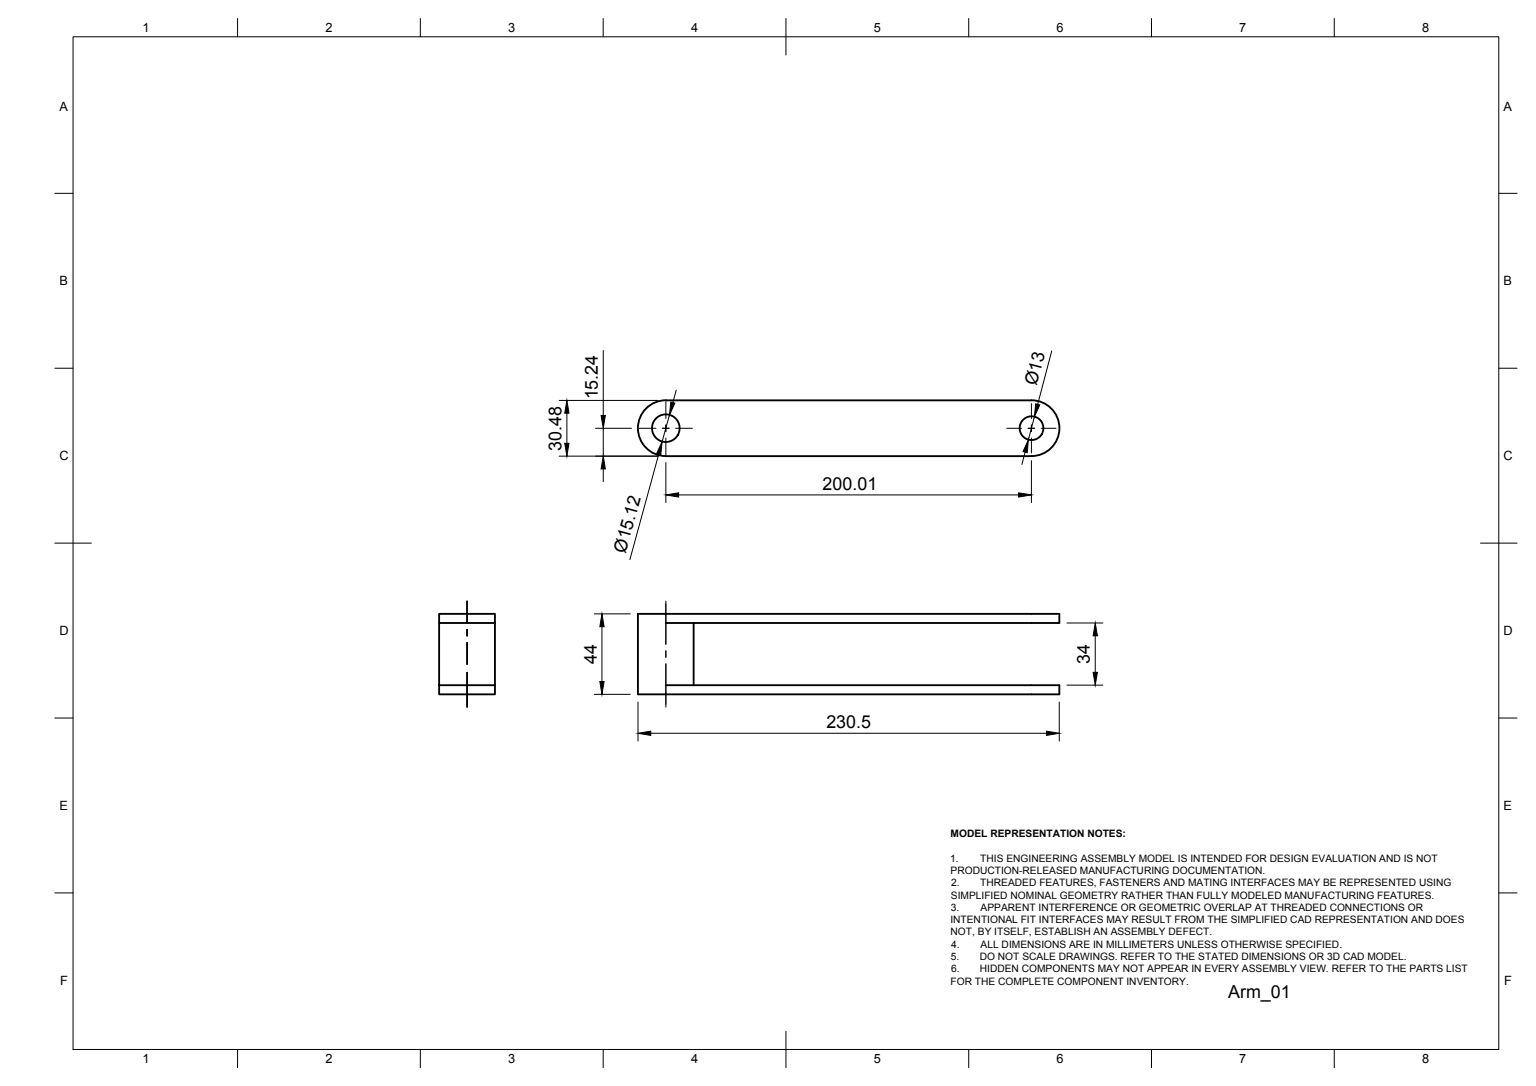
ISO-10303-21;
HEADER;
/* Generated by software containing ST-Developer
 * from STEP Tools, Inc. (www.steptools.com) 
 */

FILE_DESCRIPTION(
/* description */ (''),
/* implementation_level */ '2;1');

FILE_NAME(
/* name */ 'Arm_01.step',
/* time_stamp */ '2026-10-06T13:41:14-07:00',
/* author */ (''),
/* organization */ (''),
/* preprocessor_version */ 'ST-DEVELOPER v20.2',
/* originating_system */ 'Autodesk Translation Framework v15.15.0.0',
/* authorisation */ '');

FILE_SCHEMA (('AUTOMOTIVE_DESIGN { 1 0 10303 214 3 1 1 }'));
ENDSEC;

DATA;
#10=MECHANICAL_DESIGN_GEOMETRIC_PRESENTATION_REPRESENTATION('',(#1964),#279266);
#1946=SHAPE_REPRESENTATION_RELATIONSHIP('SRR','None',#279305,#1955);
#1955=ADVANCED_BREP_SHAPE_REPRESENTATION('',(#1973),#279261);
#1964=STYLED_ITEM('',(#279355),#1973);
#1973=MANIFOLD_SOLID_BREP('Body1',#14942);
#1996=FACE_BOUND('',#2965,.T.);
#1997=FACE_BOUND('',#2967,.T.);
#1998=FACE_BOUND('',#2968,.T.);
#1999=FACE_BOUND('',#2976,.T.);
#2000=FACE_BOUND('',#2978,.T.);
#2001=FACE_BOUND('',#2979,.T.);
#2063=PLANE('',#15478);
#2064=PLANE('',#15482);
#2065=PLANE('',#15483);
#2066=PLANE('',#15485);
#2067=PLANE('',#15493);
#2068=PLANE('',#15497);
#2069=PLANE('',#15501);
#2070=PLANE('',#15502);
#2472=FACE_OUTER_BOUND('',#2960,.T.);
#2473=FACE_OUTER_BOUND('',#2961,.T.);
#2474=FACE_OUTER_BOUND('',#2962,.T.);
#2475=FACE_OUTER_BOUND('',#2963,.T.);
#2476=FACE_OUTER_BOUND('',#2964,.T.);
#2477=FACE_OUTER_BOUND('',#2966,.T.);
#2478=FACE_OUTER_BOUND('',#2969,.T.);
#2479=FACE_OUTER_BOUND('',#2970,.T.);
#2480=FACE_OUTER_BOUND('',#2971,.T.);
#2481=FACE_OUTER_BOUND('',#2972,.T.);
#2482=FACE_OUTER_BOUND('',#2973,.T.);
#2483=FACE_OUTER_BOUND('',#2974,.T.);
#2484=FACE_OUTER_BOUND('',#2975,.T.);
#2485=FACE_OUTER_BOUND('',#2977,.T.);
#2960=EDGE_LOOP('',(#13374,#13375,#13376,#13377));
#2961=EDGE_LOOP('',(#13378,#13379,#13380,#13381));
#2962=EDGE_LOOP('',(#13382,#13383,#13384,#13385));
#2963=EDGE_LOOP('',(#13386,#13387,#13388,#13389));
#2964=EDGE_LOOP('',(#13390,#13391,#13392,#13393));
#2965=EDGE_LOOP('',(#13394));
#2966=EDGE_LOOP('',(#13395,#13396,#13397,#13398));
#2967=EDGE_LOOP('',(#13399));
#2968=EDGE_LOOP('',(#13400));
#2969=EDGE_LOOP('',(#13401,#13402,#13403,#13404));
#2970=EDGE_LOOP('',(#13405,#13406,#13407,#13408));
#2971=EDGE_LOOP('',(#13409,#13410,#13411,#13412));
#2972=EDGE_LOOP('',(#13413,#13414,#13415,#13416));
#2973=EDGE_LOOP('',(#13417,#13418,#13419,#13420));
#2974=EDGE_LOOP('',(#13421,#13422,#13423,#13424,#13425,#13426,#13427,#13428,
#13429,#13430));
#2975=EDGE_LOOP('',(#13431,#13432,#13433,#13434));
#2976=EDGE_LOOP('',(#13435));
#2977=EDGE_LOOP('',(#13436,#13437,#13438,#13439));
#2978=EDGE_LOOP('',(#13440));
#2979=EDGE_LOOP('',(#13441));
#3479=LINE('',#240456,#4007);
#3480=LINE('',#240461,#4008);
#3481=LINE('',#240463,#4009);
#3482=LINE('',#240465,#4010);
#3483=LINE('',#240466,#4011);
#3484=LINE('',#240471,#4012);
#3485=LINE('',#240475,#4013);
#3486=LINE('',#240477,#4014);
#3487=LINE('',#240478,#4015);
#3488=LINE('',#240488,#4016);
#3489=LINE('',#240493,#4017);
#3490=LINE('',#240498,#4018);
#3491=LINE('',#240500,#4019);
#3492=LINE('',#240502,#4020);
#3493=LINE('',#240503,#4021);
#3494=LINE('',#240509,#4022);
#3495=LINE('',#240512,#4023);
#3496=LINE('',#240514,#4024);
#3497=LINE('',#240515,#4025);
#3498=LINE('',#240517,#4026);
#4007=VECTOR('',#16917,6.50110764916953);
#4008=VECTOR('',#16922,10.);
#4009=VECTOR('',#16923,10.);
#4010=VECTOR('',#16924,10.);
#4011=VECTOR('',#16925,10.);
#4012=VECTOR('',#16930,10.);
#4013=VECTOR('',#16935,10.);
#4014=VECTOR('',#16936,10.);
#4015=VECTOR('',#16937,10.);
#4016=VECTOR('',#16952,7.55784864301595);
#4017=VECTOR('',#16957,6.50110764916953);
#4018=VECTOR('',#16962,10.);
#4019=VECTOR('',#16963,10.);
#4020=VECTOR('',#16964,10.);
#4021=VECTOR('',#16965,10.);
#4022=VECTOR('',#16972,10.);
#4023=VECTOR('',#16975,10.);
#4024=VECTOR('',#16976,10.);
#4025=VECTOR('',#16977,10.);
#4026=VECTOR('',#16980,15.2420394990918);
#4218=CIRCLE('',#15476,6.50110764916953);
#4219=CIRCLE('',#15477,6.50110764916953);
#4220=CIRCLE('',#15480,15.2420394990918);
#4221=CIRCLE('',#15481,15.2420394990918);
#4222=CIRCLE('',#15484,15.2420394990918);
#4223=CIRCLE('',#15486,15.2420394990918);
#4224=CIRCLE('',#15487,7.55784864301595);
#4225=CIRCLE('',#15489,7.55784864301595);
#4226=CIRCLE('',#15491,6.50110764916953);
#4227=CIRCLE('',#15492,6.50110764916953);
#4228=CIRCLE('',#15495,15.2420394990918);
#4229=CIRCLE('',#15496,15.2420394990918);
#4230=CIRCLE('',#15499,15.2420394990918);
#4231=CIRCLE('',#15500,15.2420394990918);
#6149=VERTEX_POINT('',#240453);
#6150=VERTEX_POINT('',#240455);
#6151=VERTEX_POINT('',#240459);
#6152=VERTEX_POINT('',#240460);
#6153=VERTEX_POINT('',#240462);
#6154=VERTEX_POINT('',#240464);
#6155=VERTEX_POINT('',#240468);
#6156=VERTEX_POINT('',#240470);
#6157=VERTEX_POINT('',#240474);
#6158=VERTEX_POINT('',#240476);
#6159=VERTEX_POINT('',#240483);
#6160=VERTEX_POINT('',#240486);
#6161=VERTEX_POINT('',#240490);
#6162=VERTEX_POINT('',#240492);
#6163=VERTEX_POINT('',#240496);
#6164=VERTEX_POINT('',#240497);
#6165=VERTEX_POINT('',#240499);
#6166=VERTEX_POINT('',#240501);
#6167=VERTEX_POINT('',#240505);
#6168=VERTEX_POINT('',#240507);
#6169=VERTEX_POINT('',#240511);
#6170=VERTEX_POINT('',#240513);
#8612=EDGE_CURVE('',#6149,#6149,#4218,.T.);
#8613=EDGE_CURVE('',#6149,#6150,#3479,.T.);
#8614=EDGE_CURVE('',#6150,#6150,#4219,.T.);
#8615=EDGE_CURVE('',#6151,#6152,#3480,.T.);
#8616=EDGE_CURVE('',#6151,#6153,#3481,.T.);
#8617=EDGE_CURVE('',#6153,#6154,#3482,.T.);
#8618=EDGE_CURVE('',#6152,#6154,#3483,.T.);
#8619=EDGE_CURVE('',#6155,#6151,#4220,.T.);
#8620=EDGE_CURVE('',#6155,#6156,#3484,.T.);
#8621=EDGE_CURVE('',#6156,#6153,#4221,.T.);
#8622=EDGE_CURVE('',#6157,#6155,#3485,.T.);
#8623=EDGE_CURVE('',#6157,#6158,#3486,.T.);
#8624=EDGE_CURVE('',#6158,#6156,#3487,.T.);
#8625=EDGE_CURVE('',#6158,#6154,#4222,.T.);
#8626=EDGE_CURVE('',#6152,#6157,#4223,.T.);
#8627=EDGE_CURVE('',#6159,#6159,#4224,.T.);
#8628=EDGE_CURVE('',#6160,#6160,#4225,.T.);
#8629=EDGE_CURVE('',#6160,#6159,#3488,.T.);
#8630=EDGE_CURVE('',#6161,#6161,#4226,.T.);
#8631=EDGE_CURVE('',#6161,#6162,#3489,.T.);
#8632=EDGE_CURVE('',#6162,#6162,#4227,.T.);
#8633=EDGE_CURVE('',#6163,#6164,#3490,.T.);
#8634=EDGE_CURVE('',#6164,#6165,#3491,.T.);
#8635=EDGE_CURVE('',#6166,#6165,#3492,.T.);
#8636=EDGE_CURVE('',#6163,#6166,#3493,.T.);
#8637=EDGE_CURVE('',#6167,#6163,#4228,.T.);
#8638=EDGE_CURVE('',#6168,#6166,#4229,.T.);
#8639=EDGE_CURVE('',#6167,#6168,#3494,.T.);
#8640=EDGE_CURVE('',#6169,#6167,#3495,.T.);
#8641=EDGE_CURVE('',#6170,#6168,#3496,.T.);
#8642=EDGE_CURVE('',#6169,#6170,#3497,.T.);
#8643=EDGE_CURVE('',#6158,#6170,#3498,.T.);
#8644=EDGE_CURVE('',#6165,#6170,#4230,.T.);
#8645=EDGE_CURVE('',#6164,#6169,#4231,.T.);
#13374=ORIENTED_EDGE('',*,*,#8612,.T.);
#13375=ORIENTED_EDGE('',*,*,#8613,.T.);
#13376=ORIENTED_EDGE('',*,*,#8614,.F.);
#13377=ORIENTED_EDGE('',*,*,#8613,.F.);
#13378=ORIENTED_EDGE('',*,*,#8615,.F.);
#13379=ORIENTED_EDGE('',*,*,#8616,.T.);
#13380=ORIENTED_EDGE('',*,*,#8617,.T.);
#13381=ORIENTED_EDGE('',*,*,#8618,.F.);
#13382=ORIENTED_EDGE('',*,*,#8619,.F.);
#13383=ORIENTED_EDGE('',*,*,#8620,.T.);
#13384=ORIENTED_EDGE('',*,*,#8621,.T.);
#13385=ORIENTED_EDGE('',*,*,#8616,.F.);
#13386=ORIENTED_EDGE('',*,*,#8622,.F.);
#13387=ORIENTED_EDGE('',*,*,#8623,.T.);
#13388=ORIENTED_EDGE('',*,*,#8624,.T.);
#13389=ORIENTED_EDGE('',*,*,#8620,.F.);
#13390=ORIENTED_EDGE('',*,*,#8625,.T.);
#13391=ORIENTED_EDGE('',*,*,#8617,.F.);
#13392=ORIENTED_EDGE('',*,*,#8621,.F.);
#13393=ORIENTED_EDGE('',*,*,#8624,.F.);
#13394=ORIENTED_EDGE('',*,*,#8612,.F.);
#13395=ORIENTED_EDGE('',*,*,#8626,.T.);
#13396=ORIENTED_EDGE('',*,*,#8622,.T.);
#13397=ORIENTED_EDGE('',*,*,#8619,.T.);
#13398=ORIENTED_EDGE('',*,*,#8615,.T.);
#13399=ORIENTED_EDGE('',*,*,#8614,.T.);
#13400=ORIENTED_EDGE('',*,*,#8627,.T.);
#13401=ORIENTED_EDGE('',*,*,#8628,.T.);
#13402=ORIENTED_EDGE('',*,*,#8629,.T.);
#13403=ORIENTED_EDGE('',*,*,#8627,.F.);
#13404=ORIENTED_EDGE('',*,*,#8629,.F.);
#13405=ORIENTED_EDGE('',*,*,#8630,.T.);
#13406=ORIENTED_EDGE('',*,*,#8631,.T.);
#13407=ORIENTED_EDGE('',*,*,#8632,.F.);
#13408=ORIENTED_EDGE('',*,*,#8631,.F.);
#13409=ORIENTED_EDGE('',*,*,#8633,.T.);
#13410=ORIENTED_EDGE('',*,*,#8634,.T.);
#13411=ORIENTED_EDGE('',*,*,#8635,.F.);
#13412=ORIENTED_EDGE('',*,*,#8636,.F.);
#13413=ORIENTED_EDGE('',*,*,#8637,.T.);
#13414=ORIENTED_EDGE('',*,*,#8636,.T.);
#13415=ORIENTED_EDGE('',*,*,#8638,.F.);
#13416=ORIENTED_EDGE('',*,*,#8639,.F.);
#13417=ORIENTED_EDGE('',*,*,#8640,.T.);
#13418=ORIENTED_EDGE('',*,*,#8639,.T.);
#13419=ORIENTED_EDGE('',*,*,#8641,.F.);
#13420=ORIENTED_EDGE('',*,*,#8642,.F.);
#13421=ORIENTED_EDGE('',*,*,#8623,.F.);
#13422=ORIENTED_EDGE('',*,*,#8626,.F.);
#13423=ORIENTED_EDGE('',*,*,#8618,.T.);
#13424=ORIENTED_EDGE('',*,*,#8625,.F.);
#13425=ORIENTED_EDGE('',*,*,#8643,.T.);
#13426=ORIENTED_EDGE('',*,*,#8644,.F.);
#13427=ORIENTED_EDGE('',*,*,#8634,.F.);
#13428=ORIENTED_EDGE('',*,*,#8645,.T.);
#13429=ORIENTED_EDGE('',*,*,#8642,.T.);
#13430=ORIENTED_EDGE('',*,*,#8643,.F.);
#13431=ORIENTED_EDGE('',*,*,#8644,.T.);
#13432=ORIENTED_EDGE('',*,*,#8641,.T.);
#13433=ORIENTED_EDGE('',*,*,#8638,.T.);
#13434=ORIENTED_EDGE('',*,*,#8635,.T.);
#13435=ORIENTED_EDGE('',*,*,#8632,.T.);
#13436=ORIENTED_EDGE('',*,*,#8645,.F.);
#13437=ORIENTED_EDGE('',*,*,#8633,.F.);
#13438=ORIENTED_EDGE('',*,*,#8637,.F.);
#13439=ORIENTED_EDGE('',*,*,#8640,.F.);
#13440=ORIENTED_EDGE('',*,*,#8630,.F.);
#13441=ORIENTED_EDGE('',*,*,#8628,.F.);
#14411=CYLINDRICAL_SURFACE('',#15475,6.50110764916953);
#14412=CYLINDRICAL_SURFACE('',#15479,15.2420394990918);
#14413=CYLINDRICAL_SURFACE('',#15488,7.55784864301595);
#14414=CYLINDRICAL_SURFACE('',#15490,6.50110764916953);
#14415=CYLINDRICAL_SURFACE('',#15494,15.2420394990918);
#14416=CYLINDRICAL_SURFACE('',#15498,15.2420394990918);
#14830=ADVANCED_FACE('',(#2472),#14411,.F.);
#14831=ADVANCED_FACE('',(#2473),#2063,.F.);
#14832=ADVANCED_FACE('',(#2474),#14412,.T.);
#14833=ADVANCED_FACE('',(#2475),#2064,.F.);
#14834=ADVANCED_FACE('',(#2476,#1996),#2065,.F.);
#14835=ADVANCED_FACE('',(#2477,#1997,#1998),#2066,.T.);
#14836=ADVANCED_FACE('',(#2478),#14413,.F.);
#14837=ADVANCED_FACE('',(#2479),#14414,.F.);
#14838=ADVANCED_FACE('',(#2480),#2067,.T.);
#14839=ADVANCED_FACE('',(#2481),#14415,.T.);
#14840=ADVANCED_FACE('',(#2482),#2068,.T.);
#14841=ADVANCED_FACE('',(#2483),#14416,.T.);
#14842=ADVANCED_FACE('',(#2484,#1999),#2069,.T.);
#14843=ADVANCED_FACE('',(#2485,#2000,#2001),#2070,.F.);
#14942=CLOSED_SHELL('',(#14830,#14831,#14832,#14833,#14834,#14835,#14836,
#14837,#14838,#14839,#14840,#14841,#14842,#14843));
#15474=AXIS2_PLACEMENT_3D('',#240451,#16911,#16912);
#15475=AXIS2_PLACEMENT_3D('',#240452,#16913,#16914);
#15476=AXIS2_PLACEMENT_3D('',#240454,#16915,#16916);
#15477=AXIS2_PLACEMENT_3D('',#240457,#16918,#16919);
#15478=AXIS2_PLACEMENT_3D('',#240458,#16920,#16921);
#15479=AXIS2_PLACEMENT_3D('',#240467,#16926,#16927);
#15480=AXIS2_PLACEMENT_3D('',#240469,#16928,#16929);
#15481=AXIS2_PLACEMENT_3D('',#240472,#16931,#16932);
#15482=AXIS2_PLACEMENT_3D('',#240473,#16933,#16934);
#15483=AXIS2_PLACEMENT_3D('',#240479,#16938,#16939);
#15484=AXIS2_PLACEMENT_3D('',#240480,#16940,#16941);
#15485=AXIS2_PLACEMENT_3D('',#240481,#16942,#16943);
#15486=AXIS2_PLACEMENT_3D('',#240482,#16944,#16945);
#15487=AXIS2_PLACEMENT_3D('',#240484,#16946,#16947);
#15488=AXIS2_PLACEMENT_3D('',#240485,#16948,#16949);
#15489=AXIS2_PLACEMENT_3D('',#240487,#16950,#16951);
#15490=AXIS2_PLACEMENT_3D('',#240489,#16953,#16954);
#15491=AXIS2_PLACEMENT_3D('',#240491,#16955,#16956);
#15492=AXIS2_PLACEMENT_3D('',#240494,#16958,#16959);
#15493=AXIS2_PLACEMENT_3D('',#240495,#16960,#16961);
#15494=AXIS2_PLACEMENT_3D('',#240504,#16966,#16967);
#15495=AXIS2_PLACEMENT_3D('',#240506,#16968,#16969);
#15496=AXIS2_PLACEMENT_3D('',#240508,#16970,#16971);
#15497=AXIS2_PLACEMENT_3D('',#240510,#16973,#16974);
#15498=AXIS2_PLACEMENT_3D('',#240516,#16978,#16979);
#15499=AXIS2_PLACEMENT_3D('',#240518,#16981,#16982);
#15500=AXIS2_PLACEMENT_3D('',#240519,#16983,#16984);
#15501=AXIS2_PLACEMENT_3D('',#240520,#16985,#16986);
#15502=AXIS2_PLACEMENT_3D('',#240521,#16987,#16988);
#16911=DIRECTION('axis',(0.,0.,1.));
#16912=DIRECTION('refdir',(1.,0.,0.));
#16913=DIRECTION('center_axis',(0.,1.,0.));
#16914=DIRECTION('ref_axis',(1.,0.,0.));
#16915=DIRECTION('center_axis',(0.,-1.,0.));
#16916=DIRECTION('ref_axis',(1.,0.,0.));
#16917=DIRECTION('',(0.,1.,0.));
#16918=DIRECTION('center_axis',(0.,-1.,0.));
#16919=DIRECTION('ref_axis',(1.,0.,0.));
#16920=DIRECTION('center_axis',(-0.504104280893361,0.,0.863642793048716));
#16921=DIRECTION('ref_axis',(-0.863642793048716,0.,-0.504104280893361));
#16922=DIRECTION('',(-0.863642793048716,0.,-0.504104280893361));
#16923=DIRECTION('',(0.,-1.,0.));
#16924=DIRECTION('',(-0.863642793048716,0.,-0.504104280893361));
#16925=DIRECTION('',(0.,-1.,0.));
#16926=DIRECTION('center_axis',(0.,1.,0.));
#16927=DIRECTION('ref_axis',(-0.504104280893359,0.,0.863642793048717));
#16928=DIRECTION('center_axis',(0.,1.,0.));
#16929=DIRECTION('ref_axis',(-0.504104280893359,0.,0.863642793048717));
#16930=DIRECTION('',(0.,-1.,0.));
#16931=DIRECTION('center_axis',(0.,1.,0.));
#16932=DIRECTION('ref_axis',(-0.504104280893359,0.,0.863642793048717));
#16933=DIRECTION('center_axis',(0.504104280893361,0.,-0.863642793048716));
#16934=DIRECTION('ref_axis',(0.863642793048716,0.,0.504104280893361));
#16935=DIRECTION('',(0.863642793048716,0.,0.504104280893361));
#16936=DIRECTION('',(0.,-1.,0.));
#16937=DIRECTION('',(0.863642793048716,0.,0.504104280893361));
#16938=DIRECTION('center_axis',(0.,1.,0.));
#16939=DIRECTION('ref_axis',(1.,0.,0.));
#16940=DIRECTION('center_axis',(0.,1.,0.));
#16941=DIRECTION('ref_axis',(1.,0.,0.));
#16942=DIRECTION('center_axis',(0.,1.,0.));
#16943=DIRECTION('ref_axis',(1.,0.,0.));
#16944=DIRECTION('center_axis',(0.,1.,0.));
#16945=DIRECTION('ref_axis',(0.50410428089336,0.,-0.863642793048716));
#16946=DIRECTION('center_axis',(-2.43566064310008E-53,-1.,1.62748695315959E-104));
#16947=DIRECTION('ref_axis',(1.,-2.43566064310008E-53,0.));
#16948=DIRECTION('center_axis',(0.,1.,0.));
#16949=DIRECTION('ref_axis',(1.,0.,0.));
#16950=DIRECTION('center_axis',(2.43566064310008E-53,-1.,-1.62748695315959E-104));
#16951=DIRECTION('ref_axis',(1.,2.43566064310008E-53,0.));
#16952=DIRECTION('',(0.,1.,0.));
#16953=DIRECTION('center_axis',(0.,1.,0.));
#16954=DIRECTION('ref_axis',(1.,0.,0.));
#16955=DIRECTION('center_axis',(0.,-1.,0.));
#16956=DIRECTION('ref_axis',(1.,0.,0.));
#16957=DIRECTION('',(0.,1.,0.));
#16958=DIRECTION('center_axis',(0.,-1.,0.));
#16959=DIRECTION('ref_axis',(1.,0.,0.));
#16960=DIRECTION('center_axis',(0.504104280893361,0.,-0.863642793048716));
#16961=DIRECTION('ref_axis',(-0.863642793048716,0.,-0.504104280893361));
#16962=DIRECTION('',(-0.863642793048716,0.,-0.504104280893361));
#16963=DIRECTION('',(0.,1.,0.));
#16964=DIRECTION('',(-0.863642793048716,0.,-0.504104280893361));
#16965=DIRECTION('',(0.,1.,0.));
#16966=DIRECTION('center_axis',(0.,1.,0.));
#16967=DIRECTION('ref_axis',(-0.504104280893359,0.,0.863642793048717));
#16968=DIRECTION('center_axis',(0.,1.,0.));
#16969=DIRECTION('ref_axis',(-0.504104280893359,0.,0.863642793048717));
#16970=DIRECTION('center_axis',(0.,1.,0.));
#16971=DIRECTION('ref_axis',(-0.504104280893359,0.,0.863642793048717));
#16972=DIRECTION('',(0.,1.,0.));
#16973=DIRECTION('center_axis',(-0.504104280893361,0.,0.863642793048716));
#16974=DIRECTION('ref_axis',(0.863642793048716,0.,0.504104280893361));
#16975=DIRECTION('',(0.863642793048716,0.,0.504104280893361));
#16976=DIRECTION('',(0.863642793048716,0.,0.504104280893361));
#16977=DIRECTION('',(0.,1.,0.));
#16978=DIRECTION('center_axis',(0.,1.,0.));
#16979=DIRECTION('ref_axis',(0.50410428089336,0.,-0.863642793048716));
#16980=DIRECTION('',(0.,-1.,0.));
#16981=DIRECTION('center_axis',(0.,-1.,0.));
#16982=DIRECTION('ref_axis',(1.,0.,0.));
#16983=DIRECTION('center_axis',(0.,1.,0.));
#16984=DIRECTION('ref_axis',(0.50410428089336,0.,-0.863642793048716));
#16985=DIRECTION('center_axis',(0.,1.,0.));
#16986=DIRECTION('ref_axis',(1.,0.,0.));
#16987=DIRECTION('center_axis',(0.,1.,0.));
#16988=DIRECTION('ref_axis',(1.,0.,0.));
#240451=CARTESIAN_POINT('',(0.,0.,0.));
#240452=CARTESIAN_POINT('Origin',(192.718407221598,22.,130.804360617566));
#240453=CARTESIAN_POINT('',(186.217299572429,17.,130.804360617566));
#240454=CARTESIAN_POINT('Origin',(192.718407221598,17.,130.804360617566));
#240455=CARTESIAN_POINT('',(186.217299572429,22.,130.804360617566));
#240456=CARTESIAN_POINT('',(186.217299572428,22.,130.804360617566));
#240457=CARTESIAN_POINT('Origin',(192.718407221598,22.,130.804360617566));
#240458=CARTESIAN_POINT('Origin',(200.401984582636,22.,117.640683052811));
#240459=CARTESIAN_POINT('',(200.401984582636,22.,117.640683052811));
#240460=CARTESIAN_POINT('',(27.6628184943316,22.,16.8136353382454));
#240461=CARTESIAN_POINT('',(200.401984582636,22.,117.640683052811));
#240462=CARTESIAN_POINT('',(200.401984582636,17.,117.640683052811));
#240463=CARTESIAN_POINT('',(200.401984582636,22.,117.640683052811));
#240464=CARTESIAN_POINT('',(27.6628184943316,17.,16.8136353382454));
#240465=CARTESIAN_POINT('',(200.401984582636,17.,117.640683052811));
#240466=CARTESIAN_POINT('',(27.6628184943316,22.,16.8136353382454));
#240467=CARTESIAN_POINT('Origin',(192.718407221598,22.,130.804360617566));
#240468=CARTESIAN_POINT('',(185.034829860561,22.,143.96803818232));
#240469=CARTESIAN_POINT('Origin',(192.718407221598,22.,130.804360617566));
#240470=CARTESIAN_POINT('',(185.034829860561,17.,143.96803818232));
#240471=CARTESIAN_POINT('',(185.034829860561,22.,143.96803818232));
#240472=CARTESIAN_POINT('Origin',(192.718407221598,17.,130.804360617566));
#240473=CARTESIAN_POINT('Origin',(12.2956637722558,22.,43.1409904677544));
#240474=CARTESIAN_POINT('',(12.2956637722558,22.,43.1409904677544));
#240475=CARTESIAN_POINT('',(12.2956637722558,22.,43.1409904677544));
#240476=CARTESIAN_POINT('',(12.2956637722558,17.,43.1409904677544));
#240477=CARTESIAN_POINT('',(12.2956637722558,22.,43.1409904677544));
#240478=CARTESIAN_POINT('',(12.2956637722558,17.,43.1409904677544));
#240479=CARTESIAN_POINT('Origin',(106.348824177446,17.,80.3908367602827));
#240480=CARTESIAN_POINT('Origin',(19.9792411332937,17.,29.9773129029999));
#240481=CARTESIAN_POINT('Origin',(106.348824177446,22.,80.3908367602827));
#240482=CARTESIAN_POINT('Origin',(19.9792411332937,22.,29.9773129029999));
#240483=CARTESIAN_POINT('',(12.4213924902778,22.,29.9773129029999));
#240484=CARTESIAN_POINT('Origin',(19.9792411332937,22.,29.9773129029999));
#240485=CARTESIAN_POINT('Origin',(19.9792411332937,-22.,29.9773129029999));
#240486=CARTESIAN_POINT('',(12.4213924902778,-22.,29.9773129029999));
#240487=CARTESIAN_POINT('Origin',(19.9792411332937,-22.,29.9773129029999));
#240488=CARTESIAN_POINT('',(12.4213924902778,-22.,29.9773129029999));
#240489=CARTESIAN_POINT('Origin',(192.718407221598,-22.,130.804360617566));
#240490=CARTESIAN_POINT('',(186.217299572429,-22.,130.804360617566));
#240491=CARTESIAN_POINT('Origin',(192.718407221598,-22.,130.804360617566));
#240492=CARTESIAN_POINT('',(186.217299572429,-17.,130.804360617566));
#240493=CARTESIAN_POINT('',(186.217299572428,-22.,130.804360617566));
#240494=CARTESIAN_POINT('Origin',(192.718407221598,-17.,130.804360617566));
#240495=CARTESIAN_POINT('Origin',(200.401984582636,-22.,117.640683052811));
#240496=CARTESIAN_POINT('',(200.401984582636,-22.,117.640683052811));
#240497=CARTESIAN_POINT('',(27.6628184943316,-22.,16.8136353382454));
#240498=CARTESIAN_POINT('',(200.401984582636,-22.,117.640683052811));
#240499=CARTESIAN_POINT('',(27.6628184943316,-17.,16.8136353382454));
#240500=CARTESIAN_POINT('',(27.6628184943316,-22.,16.8136353382454));
#240501=CARTESIAN_POINT('',(200.401984582636,-17.,117.640683052811));
#240502=CARTESIAN_POINT('',(200.401984582636,-17.,117.640683052811));
#240503=CARTESIAN_POINT('',(200.401984582636,-22.,117.640683052811));
#240504=CARTESIAN_POINT('Origin',(192.718407221598,-22.,130.804360617566));
#240505=CARTESIAN_POINT('',(185.034829860561,-22.,143.96803818232));
#240506=CARTESIAN_POINT('Origin',(192.718407221598,-22.,130.804360617566));
#240507=CARTESIAN_POINT('',(185.034829860561,-17.,143.96803818232));
#240508=CARTESIAN_POINT('Origin',(192.718407221598,-17.,130.804360617566));
#240509=CARTESIAN_POINT('',(185.034829860561,-22.,143.96803818232));
#240510=CARTESIAN_POINT('Origin',(12.2956637722558,-22.,43.1409904677544));
#240511=CARTESIAN_POINT('',(12.2956637722558,-22.,43.1409904677544));
#240512=CARTESIAN_POINT('',(12.2956637722558,-22.,43.1409904677544));
#240513=CARTESIAN_POINT('',(12.2956637722558,-17.,43.1409904677544));
#240514=CARTESIAN_POINT('',(12.2956637722558,-17.,43.1409904677544));
#240515=CARTESIAN_POINT('',(12.2956637722558,-22.,43.1409904677544));
#240516=CARTESIAN_POINT('Origin',(19.9792411332937,-22.,29.9773129029999));
#240517=CARTESIAN_POINT('',(12.2956637722558,-22.,43.1409904677544));
#240518=CARTESIAN_POINT('Origin',(19.9792411332937,-17.,29.9773129029999));
#240519=CARTESIAN_POINT('Origin',(19.9792411332937,-22.,29.9773129029999));
#240520=CARTESIAN_POINT('Origin',(106.348824177446,-17.,80.3908367602827));
#240521=CARTESIAN_POINT('Origin',(106.348824177446,-22.,80.3908367602827));
#279250=UNCERTAINTY_MEASURE_WITH_UNIT(LENGTH_MEASURE(0.01),#279267,
'DISTANCE_ACCURACY_VALUE',
'Maximum model space distance between geometric entities at asserted c
onnectivities');
#279255=UNCERTAINTY_MEASURE_WITH_UNIT(LENGTH_MEASURE(0.01),#279267,
'DISTANCE_ACCURACY_VALUE',
'Maximum model space distance between geometric entities at asserted c
onnectivities');
#279261=(
GEOMETRIC_REPRESENTATION_CONTEXT(3)
GLOBAL_UNCERTAINTY_ASSIGNED_CONTEXT((#279250))
GLOBAL_UNIT_ASSIGNED_CONTEXT((#279267,#279269,#279270))
REPRESENTATION_CONTEXT('','3D')
);
#279266=(
GEOMETRIC_REPRESENTATION_CONTEXT(3)
GLOBAL_UNCERTAINTY_ASSIGNED_CONTEXT((#279255))
GLOBAL_UNIT_ASSIGNED_CONTEXT((#279267,#279269,#279270))
REPRESENTATION_CONTEXT('','3D')
);
#279267=(
LENGTH_UNIT()
NAMED_UNIT(*)
SI_UNIT(.MILLI.,.METRE.)
);
#279269=(
NAMED_UNIT(*)
PLANE_ANGLE_UNIT()
SI_UNIT($,.RADIAN.)
);
#279270=(
NAMED_UNIT(*)
SI_UNIT($,.STERADIAN.)
SOLID_ANGLE_UNIT()
);
#279276=SHAPE_DEFINITION_REPRESENTATION(#279286,#279305);
#279286=PRODUCT_DEFINITION_SHAPE('',$,#279316);
#279305=SHAPE_REPRESENTATION('',(#15474),#279261);
#279310=PRODUCT_DEFINITION_CONTEXT('part definition',#279342,'design');
#279316=PRODUCT_DEFINITION('Arm_01','Arm_01',#279326,#279310);
#279326=PRODUCT_DEFINITION_FORMATION('',$,#279349);
#279342=APPLICATION_CONTEXT(
'Core Data for Automotive Mechanical Design Process');
#279343=PRODUCT_CONTEXT('part definition',#279342,'mechanical');
#279349=PRODUCT('Arm_01','Arm_01',$,(#279343));
#279355=PRESENTATION_STYLE_ASSIGNMENT((#279357));
#279357=SURFACE_STYLE_USAGE(.BOTH.,#279359);
#279359=SURFACE_SIDE_STYLE('',(#279361));
#279361=SURFACE_STYLE_FILL_AREA(#279363);
#279363=FILL_AREA_STYLE('Opaque(160,160,160)',(#279365));
#279365=FILL_AREA_STYLE_COLOUR('Opaque(160,160,160)',#279367);
#279367=COLOUR_RGB('Opaque(160,160,160)', 0.66274510, 0.83137255, 0.94901961);
ENDSEC;
END-ISO-10303-21;
